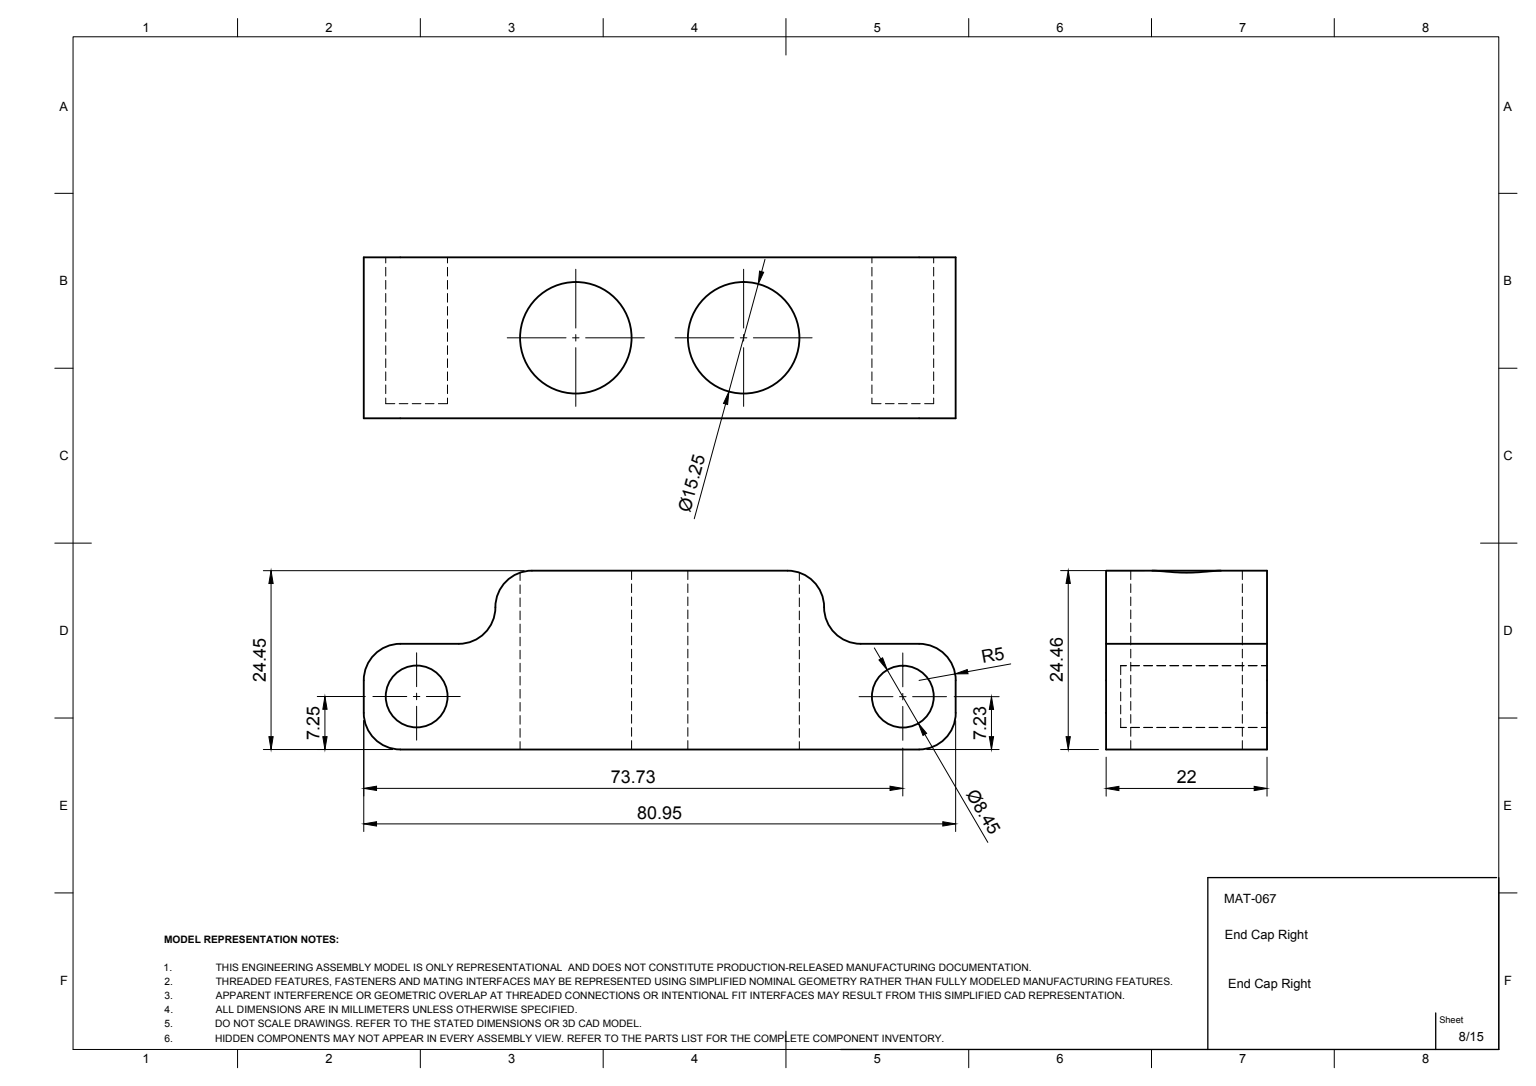
ISO-10303-21;
HEADER;
/* Generated by software containing ST-Developer
 * from STEP Tools, Inc. (www.steptools.com) 
 */

FILE_DESCRIPTION(
/* description */ ('CAx-IF Rec.Pracs.---Representation and Presentation of Product Manufa
cturing Information (PMI)---4.0---2014-10-13'),
/* implementation_level */ '2;1');

FILE_NAME(
/* name */ 'End Cap Right.step',
/* time_stamp */ '2026-10-24T16:02:03-07:00',
/* author */ (''),
/* organization */ (''),
/* preprocessor_version */ 'ST-DEVELOPER v20.2',
/* originating_system */ 'Autodesk Translation Framework v15.17.0.0',
/* authorisation */ '');

FILE_SCHEMA (('AP242_MANAGED_MODEL_BASED_3D_ENGINEERING_MIM_LF { 1 0 10303 442 2 1 4 }'));
ENDSEC;

DATA;
#10=MECHANICAL_DESIGN_GEOMETRIC_PRESENTATION_REPRESENTATION('',(#353),#6348);
#331=SHAPE_REPRESENTATION_RELATIONSHIP('SRR','None',#6482,#342);
#342=ADVANCED_BREP_SHAPE_REPRESENTATION('',(#364),#6330);
#353=STYLED_ITEM('',(#6603),#364);
#364=MANIFOLD_SOLID_BREP('Body1',#3392);
#379=B_SPLINE_CURVE_WITH_KNOTS('',3,(#5841,#5842,#5843,#5844,#5845,#5846),
 .UNSPECIFIED.,.F.,.F.,(4,2,4),(3.46797062946804,3.66737221611079,3.95578831781598),
 .UNSPECIFIED.);
#380=B_SPLINE_CURVE_WITH_KNOTS('',3,(#5847,#5848,#5849,#5850,#5851,#5852),
 .UNSPECIFIED.,.F.,.F.,(4,2,4),(3.95578831781598,4.24420441952117,4.44360600616391),
 .UNSPECIFIED.);
#381=B_SPLINE_CURVE_WITH_KNOTS('',3,(#5855,#5856,#5857,#5858,#5859,#5860,
#5861,#5862,#5863,#5864),.UNSPECIFIED.,.F.,.F.,(4,2,2,2,4),(3.46797062946804,
3.66737221611078,3.95578831781597,4.24420441952117,4.44360600616391),
 .UNSPECIFIED.);
#421=CYLINDRICAL_SURFACE('',#3690,0.004225);
#422=CYLINDRICAL_SURFACE('',#3694,0.004225);
#423=CYLINDRICAL_SURFACE('',#3717,0.005);
#424=CYLINDRICAL_SURFACE('',#3718,0.005);
#425=CYLINDRICAL_SURFACE('',#3719,0.005);
#426=CYLINDRICAL_SURFACE('',#3720,0.005);
#427=CYLINDRICAL_SURFACE('',#3725,0.007625);
#428=CYLINDRICAL_SURFACE('',#3726,0.007625);
#429=CYLINDRICAL_SURFACE('',#3727,0.005);
#430=CYLINDRICAL_SURFACE('',#3728,0.005);
#431=CYLINDRICAL_SURFACE('',#3729,0.005);
#432=CYLINDRICAL_SURFACE('',#3730,0.005);
#480=FACE_BOUND('',#960,.T.);
#481=FACE_BOUND('',#961,.T.);
#482=FACE_BOUND('',#967,.T.);
#483=FACE_BOUND('',#968,.T.);
#586=CIRCLE('',#3687,0.007625);
#587=CIRCLE('',#3688,0.007625);
#588=CIRCLE('',#3691,0.004225);
#589=CIRCLE('',#3692,0.004225);
#590=CIRCLE('',#3695,0.004225);
#591=CIRCLE('',#3696,0.004225);
#592=CIRCLE('',#3698,0.005);
#593=CIRCLE('',#3699,0.005);
#594=CIRCLE('',#3700,0.005);
#595=CIRCLE('',#3701,0.005);
#596=CIRCLE('',#3702,0.005);
#597=CIRCLE('',#3703,0.005);
#598=CIRCLE('',#3704,0.005);
#599=CIRCLE('',#3705,0.005);
#600=CIRCLE('',#3709,0.005);
#601=CIRCLE('',#3710,0.005);
#602=CIRCLE('',#3711,0.005);
#603=CIRCLE('',#3712,0.005);
#604=CIRCLE('',#3713,0.005);
#605=CIRCLE('',#3714,0.005);
#606=CIRCLE('',#3715,0.005);
#607=CIRCLE('',#3716,0.005);
#608=CIRCLE('',#3722,0.007625);
#609=CIRCLE('',#3723,0.007625);
#610=CIRCLE('',#3724,0.007625);
#770=FACE_OUTER_BOUND('',#957,.T.);
#771=FACE_OUTER_BOUND('',#958,.T.);
#772=FACE_OUTER_BOUND('',#959,.T.);
#773=FACE_OUTER_BOUND('',#962,.T.);
#774=FACE_OUTER_BOUND('',#963,.T.);
#775=FACE_OUTER_BOUND('',#964,.T.);
#776=FACE_OUTER_BOUND('',#965,.T.);
#777=FACE_OUTER_BOUND('',#966,.T.);
#778=FACE_OUTER_BOUND('',#969,.T.);
#779=FACE_OUTER_BOUND('',#970,.T.);
#780=FACE_OUTER_BOUND('',#971,.T.);
#781=FACE_OUTER_BOUND('',#972,.T.);
#782=FACE_OUTER_BOUND('',#973,.T.);
#783=FACE_OUTER_BOUND('',#974,.T.);
#784=FACE_OUTER_BOUND('',#975,.T.);
#785=FACE_OUTER_BOUND('',#976,.T.);
#786=FACE_OUTER_BOUND('',#977,.T.);
#787=FACE_OUTER_BOUND('',#978,.T.);
#788=FACE_OUTER_BOUND('',#979,.T.);
#789=FACE_OUTER_BOUND('',#980,.T.);
#790=FACE_OUTER_BOUND('',#981,.T.);
#791=FACE_OUTER_BOUND('',#982,.T.);
#957=EDGE_LOOP('',(#2723,#2724,#2725,#2726));
#958=EDGE_LOOP('',(#2727,#2728,#2729,#2730));
#959=EDGE_LOOP('',(#2731,#2732,#2733,#2734));
#960=EDGE_LOOP('',(#2735));
#961=EDGE_LOOP('',(#2736));
#962=EDGE_LOOP('',(#2737,#2738,#2739,#2740));
#963=EDGE_LOOP('',(#2741,#2742,#2743,#2744));
#964=EDGE_LOOP('',(#2745,#2746,#2747,#2748));
#965=EDGE_LOOP('',(#2749,#2750,#2751,#2752));
#966=EDGE_LOOP('',(#2753,#2754,#2755,#2756,#2757,#2758,#2759,#2760,#2761,
#2762,#2763,#2764,#2765,#2766));
#967=EDGE_LOOP('',(#2767));
#968=EDGE_LOOP('',(#2768));
#969=EDGE_LOOP('',(#2769));
#970=EDGE_LOOP('',(#2770));
#971=EDGE_LOOP('',(#2771,#2772,#2773,#2774,#2775,#2776,#2777,#2778,#2779,
#2780,#2781,#2782,#2783,#2784));
#972=EDGE_LOOP('',(#2785,#2786,#2787,#2788));
#973=EDGE_LOOP('',(#2789,#2790,#2791,#2792));
#974=EDGE_LOOP('',(#2793,#2794,#2795,#2796));
#975=EDGE_LOOP('',(#2797,#2798,#2799,#2800));
#976=EDGE_LOOP('',(#2801,#2802,#2803,#2804,#2805,#2806,#2807,#2808,#2809));
#977=EDGE_LOOP('',(#2810,#2811,#2812,#2813,#2814,#2815));
#978=EDGE_LOOP('',(#2816,#2817,#2818,#2819,#2820,#2821));
#979=EDGE_LOOP('',(#2822,#2823,#2824,#2825,#2826,#2827));
#980=EDGE_LOOP('',(#2828,#2829,#2830,#2831));
#981=EDGE_LOOP('',(#2832,#2833,#2834,#2835,#2836,#2837,#2838));
#982=EDGE_LOOP('',(#2839,#2840,#2841,#2842));
#1218=LINE('',#5733,#1451);
#1219=LINE('',#5735,#1452);
#1220=LINE('',#5737,#1453);
#1221=LINE('',#5738,#1454);
#1222=LINE('',#5742,#1455);
#1223=LINE('',#5744,#1456);
#1224=LINE('',#5746,#1457);
#1225=LINE('',#5747,#1458);
#1226=LINE('',#5751,#1459);
#1227=LINE('',#5753,#1460);
#1228=LINE('',#5755,#1461);
#1229=LINE('',#5756,#1462);
#1230=LINE('',#5764,#1463);
#1231=LINE('',#5766,#1464);
#1232=LINE('',#5768,#1465);
#1233=LINE('',#5769,#1466);
#1234=LINE('',#5774,#1467);
#1235=LINE('',#5779,#1468);
#1236=LINE('',#5781,#1469);
#1237=LINE('',#5783,#1470);
#1238=LINE('',#5784,#1471);
#1239=LINE('',#5789,#1472);
#1240=LINE('',#5794,#1473);
#1241=LINE('',#5817,#1474);
#1242=LINE('',#5827,#1475);
#1243=LINE('',#5830,#1476);
#1244=LINE('',#5832,#1477);
#1245=LINE('',#5837,#1478);
#1246=LINE('',#5840,#1479);
#1247=LINE('',#5854,#1480);
#1248=LINE('',#5866,#1481);
#1249=LINE('',#5869,#1482);
#1451=VECTOR('',#4448,1.);
#1452=VECTOR('',#4449,1.);
#1453=VECTOR('',#4450,1.);
#1454=VECTOR('',#4451,1.);
#1455=VECTOR('',#4454,1.);
#1456=VECTOR('',#4455,1.);
#1457=VECTOR('',#4456,1.);
#1458=VECTOR('',#4457,1.);
#1459=VECTOR('',#4460,1.);
#1460=VECTOR('',#4461,1.);
#1461=VECTOR('',#4462,1.);
#1462=VECTOR('',#4463,1.);
#1463=VECTOR('',#4470,1.);
#1464=VECTOR('',#4471,1.);
#1465=VECTOR('',#4472,1.);
#1466=VECTOR('',#4473,1.);
#1467=VECTOR('',#4478,0.004225);
#1468=VECTOR('',#4483,1.);
#1469=VECTOR('',#4484,1.);
#1470=VECTOR('',#4485,1.);
#1471=VECTOR('',#4486,1.);
#1472=VECTOR('',#4491,0.004225);
#1473=VECTOR('',#4496,1.);
#1474=VECTOR('',#4531,1.);
#1475=VECTOR('',#4546,1.);
#1476=VECTOR('',#4549,1.);
#1477=VECTOR('',#4550,1.);
#1478=VECTOR('',#4555,1.);
#1479=VECTOR('',#4558,0.007625);
#1480=VECTOR('',#4561,0.007625);
#1481=VECTOR('',#4564,1.);
#1482=VECTOR('',#4569,1.);
#1696=VERTEX_POINT('',#5731);
#1697=VERTEX_POINT('',#5732);
#1698=VERTEX_POINT('',#5734);
#1699=VERTEX_POINT('',#5736);
#1700=VERTEX_POINT('',#5740);
#1701=VERTEX_POINT('',#5741);
#1702=VERTEX_POINT('',#5743);
#1703=VERTEX_POINT('',#5745);
#1704=VERTEX_POINT('',#5749);
#1705=VERTEX_POINT('',#5750);
#1706=VERTEX_POINT('',#5752);
#1707=VERTEX_POINT('',#5754);
#1708=VERTEX_POINT('',#5757);
#1709=VERTEX_POINT('',#5759);
#1710=VERTEX_POINT('',#5762);
#1711=VERTEX_POINT('',#5763);
#1712=VERTEX_POINT('',#5765);
#1713=VERTEX_POINT('',#5767);
#1714=VERTEX_POINT('',#5771);
#1715=VERTEX_POINT('',#5773);
#1716=VERTEX_POINT('',#5777);
#1717=VERTEX_POINT('',#5778);
#1718=VERTEX_POINT('',#5780);
#1719=VERTEX_POINT('',#5782);
#1720=VERTEX_POINT('',#5786);
#1721=VERTEX_POINT('',#5788);
#1722=VERTEX_POINT('',#5792);
#1723=VERTEX_POINT('',#5793);
#1724=VERTEX_POINT('',#5795);
#1725=VERTEX_POINT('',#5802);
#1726=VERTEX_POINT('',#5812);
#1727=VERTEX_POINT('',#5814);
#1728=VERTEX_POINT('',#5816);
#1729=VERTEX_POINT('',#5818);
#1730=VERTEX_POINT('',#5826);
#1731=VERTEX_POINT('',#5828);
#1732=VERTEX_POINT('',#5831);
#1733=VERTEX_POINT('',#5833);
#1734=VERTEX_POINT('',#5835);
#1735=VERTEX_POINT('',#5839);
#2060=EDGE_CURVE('',#1696,#1697,#1218,.T.);
#2061=EDGE_CURVE('',#1698,#1697,#1219,.T.);
#2062=EDGE_CURVE('',#1699,#1698,#1220,.T.);
#2063=EDGE_CURVE('',#1696,#1699,#1221,.F.);
#2064=EDGE_CURVE('',#1700,#1701,#1222,.T.);
#2065=EDGE_CURVE('',#1702,#1700,#1223,.F.);
#2066=EDGE_CURVE('',#1702,#1703,#1224,.T.);
#2067=EDGE_CURVE('',#1701,#1703,#1225,.T.);
#2068=EDGE_CURVE('',#1704,#1705,#1226,.T.);
#2069=EDGE_CURVE('',#1706,#1705,#1227,.F.);
#2070=EDGE_CURVE('',#1707,#1706,#1228,.T.);
#2071=EDGE_CURVE('',#1704,#1707,#1229,.T.);
#2072=EDGE_CURVE('',#1708,#1708,#586,.T.);
#2073=EDGE_CURVE('',#1709,#1709,#587,.T.);
#2074=EDGE_CURVE('',#1710,#1711,#1230,.T.);
#2075=EDGE_CURVE('',#1712,#1711,#1231,.F.);
#2076=EDGE_CURVE('',#1713,#1712,#1232,.T.);
#2077=EDGE_CURVE('',#1710,#1713,#1233,.T.);
#2078=EDGE_CURVE('',#1714,#1714,#588,.T.);
#2079=EDGE_CURVE('',#1714,#1715,#1234,.T.);
#2080=EDGE_CURVE('',#1715,#1715,#589,.T.);
#2081=EDGE_CURVE('',#1716,#1717,#1235,.T.);
#2082=EDGE_CURVE('',#1718,#1716,#1236,.F.);
#2083=EDGE_CURVE('',#1718,#1719,#1237,.T.);
#2084=EDGE_CURVE('',#1717,#1719,#1238,.T.);
#2085=EDGE_CURVE('',#1720,#1720,#590,.T.);
#2086=EDGE_CURVE('',#1720,#1721,#1239,.T.);
#2087=EDGE_CURVE('',#1721,#1721,#591,.T.);
#2088=EDGE_CURVE('',#1722,#1723,#1240,.T.);
#2089=EDGE_CURVE('',#1724,#1722,#592,.F.);
#2090=EDGE_CURVE('',#1719,#1724,#593,.T.);
#2091=EDGE_CURVE('',#1703,#1718,#594,.F.);
#2092=EDGE_CURVE('',#1707,#1702,#595,.F.);
#2093=EDGE_CURVE('',#1713,#1706,#596,.F.);
#2094=EDGE_CURVE('',#1697,#1712,#597,.F.);
#2095=EDGE_CURVE('',#1725,#1696,#598,.T.);
#2096=EDGE_CURVE('',#1723,#1725,#599,.F.);
#2097=EDGE_CURVE('',#1711,#1698,#600,.T.);
#2098=EDGE_CURVE('',#1705,#1710,#601,.T.);
#2099=EDGE_CURVE('',#1700,#1704,#602,.T.);
#2100=EDGE_CURVE('',#1716,#1701,#603,.T.);
#2101=EDGE_CURVE('',#1726,#1717,#604,.F.);
#2102=EDGE_CURVE('',#1727,#1726,#605,.T.);
#2103=EDGE_CURVE('',#1727,#1728,#1241,.T.);
#2104=EDGE_CURVE('',#1729,#1728,#606,.T.);
#2105=EDGE_CURVE('',#1699,#1729,#607,.F.);
#2106=EDGE_CURVE('',#1730,#1727,#1242,.F.);
#2107=EDGE_CURVE('',#1730,#1731,#608,.T.);
#2108=EDGE_CURVE('',#1722,#1731,#1243,.F.);
#2109=EDGE_CURVE('',#1732,#1723,#1244,.T.);
#2110=EDGE_CURVE('',#1732,#1733,#609,.T.);
#2111=EDGE_CURVE('',#1733,#1734,#610,.T.);
#2112=EDGE_CURVE('',#1728,#1734,#1245,.T.);
#2113=EDGE_CURVE('',#1709,#1735,#1246,.T.);
#2114=EDGE_CURVE('',#1731,#1735,#379,.T.);
#2115=EDGE_CURVE('',#1735,#1730,#380,.T.);
#2116=EDGE_CURVE('',#1708,#1733,#1247,.T.);
#2117=EDGE_CURVE('',#1734,#1732,#381,.T.);
#2118=EDGE_CURVE('',#1725,#1729,#1248,.F.);
#2119=EDGE_CURVE('',#1726,#1724,#1249,.T.);
#2723=ORIENTED_EDGE('',*,*,#2060,.T.);
#2724=ORIENTED_EDGE('',*,*,#2061,.F.);
#2725=ORIENTED_EDGE('',*,*,#2062,.F.);
#2726=ORIENTED_EDGE('',*,*,#2063,.F.);
#2727=ORIENTED_EDGE('',*,*,#2064,.F.);
#2728=ORIENTED_EDGE('',*,*,#2065,.F.);
#2729=ORIENTED_EDGE('',*,*,#2066,.T.);
#2730=ORIENTED_EDGE('',*,*,#2067,.F.);
#2731=ORIENTED_EDGE('',*,*,#2068,.T.);
#2732=ORIENTED_EDGE('',*,*,#2069,.F.);
#2733=ORIENTED_EDGE('',*,*,#2070,.F.);
#2734=ORIENTED_EDGE('',*,*,#2071,.F.);
#2735=ORIENTED_EDGE('',*,*,#2072,.F.);
#2736=ORIENTED_EDGE('',*,*,#2073,.F.);
#2737=ORIENTED_EDGE('',*,*,#2074,.T.);
#2738=ORIENTED_EDGE('',*,*,#2075,.F.);
#2739=ORIENTED_EDGE('',*,*,#2076,.F.);
#2740=ORIENTED_EDGE('',*,*,#2077,.F.);
#2741=ORIENTED_EDGE('',*,*,#2078,.F.);
#2742=ORIENTED_EDGE('',*,*,#2079,.T.);
#2743=ORIENTED_EDGE('',*,*,#2080,.T.);
#2744=ORIENTED_EDGE('',*,*,#2079,.F.);
#2745=ORIENTED_EDGE('',*,*,#2081,.F.);
#2746=ORIENTED_EDGE('',*,*,#2082,.F.);
#2747=ORIENTED_EDGE('',*,*,#2083,.T.);
#2748=ORIENTED_EDGE('',*,*,#2084,.F.);
#2749=ORIENTED_EDGE('',*,*,#2085,.F.);
#2750=ORIENTED_EDGE('',*,*,#2086,.T.);
#2751=ORIENTED_EDGE('',*,*,#2087,.T.);
#2752=ORIENTED_EDGE('',*,*,#2086,.F.);
#2753=ORIENTED_EDGE('',*,*,#2088,.F.);
#2754=ORIENTED_EDGE('',*,*,#2089,.F.);
#2755=ORIENTED_EDGE('',*,*,#2090,.F.);
#2756=ORIENTED_EDGE('',*,*,#2083,.F.);
#2757=ORIENTED_EDGE('',*,*,#2091,.F.);
#2758=ORIENTED_EDGE('',*,*,#2066,.F.);
#2759=ORIENTED_EDGE('',*,*,#2092,.F.);
#2760=ORIENTED_EDGE('',*,*,#2070,.T.);
#2761=ORIENTED_EDGE('',*,*,#2093,.F.);
#2762=ORIENTED_EDGE('',*,*,#2076,.T.);
#2763=ORIENTED_EDGE('',*,*,#2094,.F.);
#2764=ORIENTED_EDGE('',*,*,#2060,.F.);
#2765=ORIENTED_EDGE('',*,*,#2095,.F.);
#2766=ORIENTED_EDGE('',*,*,#2096,.F.);
#2767=ORIENTED_EDGE('',*,*,#2080,.F.);
#2768=ORIENTED_EDGE('',*,*,#2087,.F.);
#2769=ORIENTED_EDGE('',*,*,#2085,.T.);
#2770=ORIENTED_EDGE('',*,*,#2078,.T.);
#2771=ORIENTED_EDGE('',*,*,#2062,.T.);
#2772=ORIENTED_EDGE('',*,*,#2097,.F.);
#2773=ORIENTED_EDGE('',*,*,#2074,.F.);
#2774=ORIENTED_EDGE('',*,*,#2098,.F.);
#2775=ORIENTED_EDGE('',*,*,#2068,.F.);
#2776=ORIENTED_EDGE('',*,*,#2099,.F.);
#2777=ORIENTED_EDGE('',*,*,#2064,.T.);
#2778=ORIENTED_EDGE('',*,*,#2100,.F.);
#2779=ORIENTED_EDGE('',*,*,#2081,.T.);
#2780=ORIENTED_EDGE('',*,*,#2101,.F.);
#2781=ORIENTED_EDGE('',*,*,#2102,.F.);
#2782=ORIENTED_EDGE('',*,*,#2103,.T.);
#2783=ORIENTED_EDGE('',*,*,#2104,.F.);
#2784=ORIENTED_EDGE('',*,*,#2105,.F.);
#2785=ORIENTED_EDGE('',*,*,#2100,.T.);
#2786=ORIENTED_EDGE('',*,*,#2067,.T.);
#2787=ORIENTED_EDGE('',*,*,#2091,.T.);
#2788=ORIENTED_EDGE('',*,*,#2082,.T.);
#2789=ORIENTED_EDGE('',*,*,#2099,.T.);
#2790=ORIENTED_EDGE('',*,*,#2071,.T.);
#2791=ORIENTED_EDGE('',*,*,#2092,.T.);
#2792=ORIENTED_EDGE('',*,*,#2065,.T.);
#2793=ORIENTED_EDGE('',*,*,#2098,.T.);
#2794=ORIENTED_EDGE('',*,*,#2077,.T.);
#2795=ORIENTED_EDGE('',*,*,#2093,.T.);
#2796=ORIENTED_EDGE('',*,*,#2069,.T.);
#2797=ORIENTED_EDGE('',*,*,#2097,.T.);
#2798=ORIENTED_EDGE('',*,*,#2061,.T.);
#2799=ORIENTED_EDGE('',*,*,#2094,.T.);
#2800=ORIENTED_EDGE('',*,*,#2075,.T.);
#2801=ORIENTED_EDGE('',*,*,#2103,.F.);
#2802=ORIENTED_EDGE('',*,*,#2106,.F.);
#2803=ORIENTED_EDGE('',*,*,#2107,.T.);
#2804=ORIENTED_EDGE('',*,*,#2108,.F.);
#2805=ORIENTED_EDGE('',*,*,#2088,.T.);
#2806=ORIENTED_EDGE('',*,*,#2109,.F.);
#2807=ORIENTED_EDGE('',*,*,#2110,.T.);
#2808=ORIENTED_EDGE('',*,*,#2111,.T.);
#2809=ORIENTED_EDGE('',*,*,#2112,.F.);
#2810=ORIENTED_EDGE('',*,*,#2073,.T.);
#2811=ORIENTED_EDGE('',*,*,#2113,.T.);
#2812=ORIENTED_EDGE('',*,*,#2114,.F.);
#2813=ORIENTED_EDGE('',*,*,#2107,.F.);
#2814=ORIENTED_EDGE('',*,*,#2115,.F.);
#2815=ORIENTED_EDGE('',*,*,#2113,.F.);
#2816=ORIENTED_EDGE('',*,*,#2072,.T.);
#2817=ORIENTED_EDGE('',*,*,#2116,.T.);
#2818=ORIENTED_EDGE('',*,*,#2110,.F.);
#2819=ORIENTED_EDGE('',*,*,#2117,.F.);
#2820=ORIENTED_EDGE('',*,*,#2111,.F.);
#2821=ORIENTED_EDGE('',*,*,#2116,.F.);
#2822=ORIENTED_EDGE('',*,*,#2112,.T.);
#2823=ORIENTED_EDGE('',*,*,#2117,.T.);
#2824=ORIENTED_EDGE('',*,*,#2109,.T.);
#2825=ORIENTED_EDGE('',*,*,#2096,.T.);
#2826=ORIENTED_EDGE('',*,*,#2118,.T.);
#2827=ORIENTED_EDGE('',*,*,#2104,.T.);
#2828=ORIENTED_EDGE('',*,*,#2105,.T.);
#2829=ORIENTED_EDGE('',*,*,#2118,.F.);
#2830=ORIENTED_EDGE('',*,*,#2095,.T.);
#2831=ORIENTED_EDGE('',*,*,#2063,.T.);
#2832=ORIENTED_EDGE('',*,*,#2119,.T.);
#2833=ORIENTED_EDGE('',*,*,#2089,.T.);
#2834=ORIENTED_EDGE('',*,*,#2108,.T.);
#2835=ORIENTED_EDGE('',*,*,#2114,.T.);
#2836=ORIENTED_EDGE('',*,*,#2115,.T.);
#2837=ORIENTED_EDGE('',*,*,#2106,.T.);
#2838=ORIENTED_EDGE('',*,*,#2102,.T.);
#2839=ORIENTED_EDGE('',*,*,#2101,.T.);
#2840=ORIENTED_EDGE('',*,*,#2084,.T.);
#2841=ORIENTED_EDGE('',*,*,#2090,.T.);
#2842=ORIENTED_EDGE('',*,*,#2119,.F.);
#3177=PLANE('',#3684);
#3178=PLANE('',#3685);
#3179=PLANE('',#3686);
#3180=PLANE('',#3689);
#3181=PLANE('',#3693);
#3182=PLANE('',#3697);
#3183=PLANE('',#3706);
#3184=PLANE('',#3707);
#3185=PLANE('',#3708);
#3186=PLANE('',#3721);
#3293=ADVANCED_FACE('',(#770),#3177,.T.);
#3294=ADVANCED_FACE('',(#771),#3178,.T.);
#3295=ADVANCED_FACE('',(#772,#480,#481),#3179,.F.);
#3296=ADVANCED_FACE('',(#773),#3180,.F.);
#3297=ADVANCED_FACE('',(#774),#421,.F.);
#3298=ADVANCED_FACE('',(#775),#3181,.T.);
#3299=ADVANCED_FACE('',(#776),#422,.F.);
#3300=ADVANCED_FACE('',(#777,#482,#483),#3182,.F.);
#3301=ADVANCED_FACE('',(#778),#3183,.F.);
#3302=ADVANCED_FACE('',(#779),#3184,.F.);
#3303=ADVANCED_FACE('',(#780),#3185,.T.);
#3304=ADVANCED_FACE('',(#781),#423,.T.);
#3305=ADVANCED_FACE('',(#782),#424,.T.);
#3306=ADVANCED_FACE('',(#783),#425,.T.);
#3307=ADVANCED_FACE('',(#784),#426,.T.);
#3308=ADVANCED_FACE('',(#785),#3186,.T.);
#3309=ADVANCED_FACE('',(#786),#427,.F.);
#3310=ADVANCED_FACE('',(#787),#428,.F.);
#3311=ADVANCED_FACE('',(#788),#429,.T.);
#3312=ADVANCED_FACE('',(#789),#430,.F.);
#3313=ADVANCED_FACE('',(#790),#431,.T.);
#3314=ADVANCED_FACE('',(#791),#432,.F.);
#3392=CLOSED_SHELL('',(#3293,#3294,#3295,#3296,#3297,#3298,#3299,#3300,
#3301,#3302,#3303,#3304,#3305,#3306,#3307,#3308,#3309,#3310,#3311,#3312,
#3313,#3314));
#3683=AXIS2_PLACEMENT_3D('',#5729,#4444,#4445);
#3684=AXIS2_PLACEMENT_3D('',#5730,#4446,#4447);
#3685=AXIS2_PLACEMENT_3D('',#5739,#4452,#4453);
#3686=AXIS2_PLACEMENT_3D('',#5748,#4458,#4459);
#3687=AXIS2_PLACEMENT_3D('',#5758,#4464,#4465);
#3688=AXIS2_PLACEMENT_3D('',#5760,#4466,#4467);
#3689=AXIS2_PLACEMENT_3D('',#5761,#4468,#4469);
#3690=AXIS2_PLACEMENT_3D('',#5770,#4474,#4475);
#3691=AXIS2_PLACEMENT_3D('',#5772,#4476,#4477);
#3692=AXIS2_PLACEMENT_3D('',#5775,#4479,#4480);
#3693=AXIS2_PLACEMENT_3D('',#5776,#4481,#4482);
#3694=AXIS2_PLACEMENT_3D('',#5785,#4487,#4488);
#3695=AXIS2_PLACEMENT_3D('',#5787,#4489,#4490);
#3696=AXIS2_PLACEMENT_3D('',#5790,#4492,#4493);
#3697=AXIS2_PLACEMENT_3D('',#5791,#4494,#4495);
#3698=AXIS2_PLACEMENT_3D('',#5796,#4497,#4498);
#3699=AXIS2_PLACEMENT_3D('',#5797,#4499,#4500);
#3700=AXIS2_PLACEMENT_3D('',#5798,#4501,#4502);
#3701=AXIS2_PLACEMENT_3D('',#5799,#4503,#4504);
#3702=AXIS2_PLACEMENT_3D('',#5800,#4505,#4506);
#3703=AXIS2_PLACEMENT_3D('',#5801,#4507,#4508);
#3704=AXIS2_PLACEMENT_3D('',#5803,#4509,#4510);
#3705=AXIS2_PLACEMENT_3D('',#5804,#4511,#4512);
#3706=AXIS2_PLACEMENT_3D('',#5805,#4513,#4514);
#3707=AXIS2_PLACEMENT_3D('',#5806,#4515,#4516);
#3708=AXIS2_PLACEMENT_3D('',#5807,#4517,#4518);
#3709=AXIS2_PLACEMENT_3D('',#5808,#4519,#4520);
#3710=AXIS2_PLACEMENT_3D('',#5809,#4521,#4522);
#3711=AXIS2_PLACEMENT_3D('',#5810,#4523,#4524);
#3712=AXIS2_PLACEMENT_3D('',#5811,#4525,#4526);
#3713=AXIS2_PLACEMENT_3D('',#5813,#4527,#4528);
#3714=AXIS2_PLACEMENT_3D('',#5815,#4529,#4530);
#3715=AXIS2_PLACEMENT_3D('',#5819,#4532,#4533);
#3716=AXIS2_PLACEMENT_3D('',#5820,#4534,#4535);
#3717=AXIS2_PLACEMENT_3D('',#5821,#4536,#4537);
#3718=AXIS2_PLACEMENT_3D('',#5822,#4538,#4539);
#3719=AXIS2_PLACEMENT_3D('',#5823,#4540,#4541);
#3720=AXIS2_PLACEMENT_3D('',#5824,#4542,#4543);
#3721=AXIS2_PLACEMENT_3D('',#5825,#4544,#4545);
#3722=AXIS2_PLACEMENT_3D('',#5829,#4547,#4548);
#3723=AXIS2_PLACEMENT_3D('',#5834,#4551,#4552);
#3724=AXIS2_PLACEMENT_3D('',#5836,#4553,#4554);
#3725=AXIS2_PLACEMENT_3D('',#5838,#4556,#4557);
#3726=AXIS2_PLACEMENT_3D('',#5853,#4559,#4560);
#3727=AXIS2_PLACEMENT_3D('',#5865,#4562,#4563);
#3728=AXIS2_PLACEMENT_3D('',#5867,#4565,#4566);
#3729=AXIS2_PLACEMENT_3D('',#5868,#4567,#4568);
#3730=AXIS2_PLACEMENT_3D('',#5870,#4570,#4571);
#4444=DIRECTION('axis',(0.,0.,1.));
#4445=DIRECTION('refdir',(1.,0.,0.));
#4446=DIRECTION('center_axis',(0.,-1.,8.57182693503055E-17));
#4447=DIRECTION('ref_axis',(0.,-8.57182693503055E-17,-1.));
#4448=DIRECTION('',(0.,-8.57182693503055E-17,-1.));
#4449=DIRECTION('',(-1.,0.,0.));
#4450=DIRECTION('',(0.,-8.57182693503055E-17,-1.));
#4451=DIRECTION('',(-1.,0.,0.));
#4452=DIRECTION('center_axis',(0.,0.,1.));
#4453=DIRECTION('ref_axis',(-1.,0.,0.));
#4454=DIRECTION('',(0.,-1.,0.));
#4455=DIRECTION('',(-1.,0.,0.));
#4456=DIRECTION('',(0.,-1.,0.));
#4457=DIRECTION('',(-1.,0.,0.));
#4458=DIRECTION('center_axis',(0.,-1.,6.42887020127291E-17));
#4459=DIRECTION('ref_axis',(0.,-6.42887020127291E-17,-1.));
#4460=DIRECTION('',(0.,-6.42887020127291E-17,-1.));
#4461=DIRECTION('',(-1.,0.,0.));
#4462=DIRECTION('',(0.,-6.42887020127291E-17,-1.));
#4463=DIRECTION('',(-1.,0.,0.));
#4464=DIRECTION('center_axis',(0.,1.,-6.42887020127291E-17));
#4465=DIRECTION('ref_axis',(0.,-6.42887020127291E-17,-1.));
#4466=DIRECTION('center_axis',(0.,1.,-6.42887020127291E-17));
#4467=DIRECTION('ref_axis',(0.,-6.42887020127291E-17,-1.));
#4468=DIRECTION('center_axis',(0.,0.,1.));
#4469=DIRECTION('ref_axis',(-1.,0.,0.));
#4470=DIRECTION('',(0.,-1.,0.));
#4471=DIRECTION('',(-1.,0.,0.));
#4472=DIRECTION('',(0.,-1.,0.));
#4473=DIRECTION('',(-1.,0.,0.));
#4474=DIRECTION('center_axis',(-1.,0.,0.));
#4475=DIRECTION('ref_axis',(0.,0.,-1.));
#4476=DIRECTION('center_axis',(-1.,0.,0.));
#4477=DIRECTION('ref_axis',(0.,0.,1.));
#4478=DIRECTION('',(-1.,0.,0.));
#4479=DIRECTION('center_axis',(-1.,0.,0.));
#4480=DIRECTION('ref_axis',(0.,0.,1.));
#4481=DIRECTION('center_axis',(0.,-1.,8.57182693503055E-17));
#4482=DIRECTION('ref_axis',(0.,-8.57182693503055E-17,-1.));
#4483=DIRECTION('',(0.,-8.57182693503055E-17,-1.));
#4484=DIRECTION('',(-1.,0.,0.));
#4485=DIRECTION('',(0.,-8.57182693503055E-17,-1.));
#4486=DIRECTION('',(-1.,0.,0.));
#4487=DIRECTION('center_axis',(-1.,0.,0.));
#4488=DIRECTION('ref_axis',(0.,0.,-1.));
#4489=DIRECTION('center_axis',(-1.,0.,0.));
#4490=DIRECTION('ref_axis',(0.,0.,1.));
#4491=DIRECTION('',(-1.,0.,0.));
#4492=DIRECTION('center_axis',(-1.,0.,0.));
#4493=DIRECTION('ref_axis',(0.,0.,1.));
#4494=DIRECTION('center_axis',(1.,0.,0.));
#4495=DIRECTION('ref_axis',(0.,-1.,0.));
#4496=DIRECTION('',(0.,-8.57182693503055E-17,-1.));
#4497=DIRECTION('center_axis',(-1.,0.,0.));
#4498=DIRECTION('ref_axis',(0.,0.,1.));
#4499=DIRECTION('center_axis',(-1.,0.,0.));
#4500=DIRECTION('ref_axis',(0.,0.,1.));
#4501=DIRECTION('center_axis',(-1.,0.,0.));
#4502=DIRECTION('ref_axis',(0.,0.,1.));
#4503=DIRECTION('center_axis',(-1.,0.,0.));
#4504=DIRECTION('ref_axis',(0.,0.,1.));
#4505=DIRECTION('center_axis',(-1.,0.,0.));
#4506=DIRECTION('ref_axis',(0.,0.,1.));
#4507=DIRECTION('center_axis',(-1.,0.,0.));
#4508=DIRECTION('ref_axis',(0.,0.,1.));
#4509=DIRECTION('center_axis',(-1.,0.,0.));
#4510=DIRECTION('ref_axis',(0.,0.,1.));
#4511=DIRECTION('center_axis',(-1.,0.,0.));
#4512=DIRECTION('ref_axis',(0.,0.,1.));
#4513=DIRECTION('center_axis',(1.,0.,0.));
#4514=DIRECTION('ref_axis',(0.,-1.,0.));
#4515=DIRECTION('center_axis',(1.,0.,0.));
#4516=DIRECTION('ref_axis',(0.,-1.,0.));
#4517=DIRECTION('center_axis',(1.,0.,0.));
#4518=DIRECTION('ref_axis',(0.,-1.,0.));
#4519=DIRECTION('center_axis',(-1.,0.,0.));
#4520=DIRECTION('ref_axis',(0.,0.,1.));
#4521=DIRECTION('center_axis',(-1.,0.,0.));
#4522=DIRECTION('ref_axis',(0.,0.,1.));
#4523=DIRECTION('center_axis',(-1.,0.,0.));
#4524=DIRECTION('ref_axis',(0.,0.,1.));
#4525=DIRECTION('center_axis',(-1.,0.,0.));
#4526=DIRECTION('ref_axis',(0.,0.,1.));
#4527=DIRECTION('center_axis',(-1.,0.,0.));
#4528=DIRECTION('ref_axis',(0.,0.,1.));
#4529=DIRECTION('center_axis',(-1.,0.,0.));
#4530=DIRECTION('ref_axis',(0.,0.,1.));
#4531=DIRECTION('',(0.,-8.57182693503055E-17,-1.));
#4532=DIRECTION('center_axis',(-1.,0.,0.));
#4533=DIRECTION('ref_axis',(0.,0.,1.));
#4534=DIRECTION('center_axis',(-1.,0.,0.));
#4535=DIRECTION('ref_axis',(0.,0.,1.));
#4536=DIRECTION('center_axis',(-1.,0.,0.));
#4537=DIRECTION('ref_axis',(0.,0.,-1.));
#4538=DIRECTION('center_axis',(1.,0.,0.));
#4539=DIRECTION('ref_axis',(0.,0.,1.));
#4540=DIRECTION('center_axis',(-1.,0.,0.));
#4541=DIRECTION('ref_axis',(0.,0.,-1.));
#4542=DIRECTION('center_axis',(1.,0.,0.));
#4543=DIRECTION('ref_axis',(0.,0.,1.));
#4544=DIRECTION('center_axis',(0.,-1.,8.57182693503055E-17));
#4545=DIRECTION('ref_axis',(-1.,0.,0.));
#4546=DIRECTION('',(-1.,0.,0.));
#4547=DIRECTION('center_axis',(0.,1.,-8.57182693503055E-17));
#4548=DIRECTION('ref_axis',(0.,-8.57182693503055E-17,-1.));
#4549=DIRECTION('',(-1.,0.,0.));
#4550=DIRECTION('',(-1.,0.,0.));
#4551=DIRECTION('center_axis',(0.,1.,-8.57182693503055E-17));
#4552=DIRECTION('ref_axis',(0.,-8.57182693503055E-17,-1.));
#4553=DIRECTION('center_axis',(0.,1.,-8.57182693503055E-17));
#4554=DIRECTION('ref_axis',(0.,-8.57182693503055E-17,-1.));
#4555=DIRECTION('',(-1.,0.,0.));
#4556=DIRECTION('center_axis',(0.,-1.,8.57182693503055E-17));
#4557=DIRECTION('ref_axis',(0.,-8.57182693503055E-17,-1.));
#4558=DIRECTION('',(0.,-1.,8.57182693503055E-17));
#4559=DIRECTION('center_axis',(0.,-1.,8.57182693503055E-17));
#4560=DIRECTION('ref_axis',(0.,-8.57182693503055E-17,-1.));
#4561=DIRECTION('',(0.,-1.,8.57182693503055E-17));
#4562=DIRECTION('center_axis',(1.,0.,0.));
#4563=DIRECTION('ref_axis',(0.,0.,1.));
#4564=DIRECTION('',(-1.,0.,0.));
#4565=DIRECTION('center_axis',(-1.,0.,0.));
#4566=DIRECTION('ref_axis',(0.,0.,-1.));
#4567=DIRECTION('center_axis',(-1.,0.,0.));
#4568=DIRECTION('ref_axis',(0.,0.,-1.));
#4569=DIRECTION('',(-1.,0.,0.));
#4570=DIRECTION('center_axis',(1.,0.,0.));
#4571=DIRECTION('ref_axis',(0.,0.,1.));
#5729=CARTESIAN_POINT('',(0.,0.,0.));
#5730=CARTESIAN_POINT('Origin',(0.06655,-0.0172,0.02565));
#5731=CARTESIAN_POINT('',(0.04655,-0.0172,-0.001825));
#5732=CARTESIAN_POINT('',(0.04655,-0.0172,-0.009825));
#5733=CARTESIAN_POINT('',(0.04655,-0.0172,0.02565));
#5734=CARTESIAN_POINT('',(0.06855,-0.0172,-0.009825));
#5735=CARTESIAN_POINT('',(0.04655,-0.0172,-0.009825));
#5736=CARTESIAN_POINT('',(0.06855,-0.0172,-0.001825));
#5737=CARTESIAN_POINT('',(0.06855,-0.0172,0.02565));
#5738=CARTESIAN_POINT('',(0.06655,-0.0172,-0.001825));
#5739=CARTESIAN_POINT('Origin',(0.06655,-0.009975,0.066125));
#5740=CARTESIAN_POINT('',(0.06855,-0.00775,0.066125));
#5741=CARTESIAN_POINT('',(0.06855,-0.0122,0.066125));
#5742=CARTESIAN_POINT('',(0.06855,-0.009975,0.066125));
#5743=CARTESIAN_POINT('',(0.04655,-0.00775,0.066125));
#5744=CARTESIAN_POINT('',(0.06855,-0.00775,0.066125));
#5745=CARTESIAN_POINT('',(0.04655,-0.0122,0.066125));
#5746=CARTESIAN_POINT('',(0.04655,-0.009975,0.066125));
#5747=CARTESIAN_POINT('',(0.06655,-0.0122,0.066125));
#5748=CARTESIAN_POINT('Origin',(0.06655,-0.00275,0.02565));
#5749=CARTESIAN_POINT('',(0.06855,-0.00275,0.061125));
#5750=CARTESIAN_POINT('',(0.06855,-0.00275,-0.009825));
#5751=CARTESIAN_POINT('',(0.06855,-0.00275,0.02565));
#5752=CARTESIAN_POINT('',(0.04655,-0.00275,-0.009825));
#5753=CARTESIAN_POINT('',(0.06655,-0.00275,-0.009825));
#5754=CARTESIAN_POINT('',(0.04655,-0.00275,0.061125));
#5755=CARTESIAN_POINT('',(0.04655,-0.00275,0.02565));
#5756=CARTESIAN_POINT('',(0.04655,-0.00275,0.061125));
#5757=CARTESIAN_POINT('',(0.05755,-0.00275,0.0218));
#5758=CARTESIAN_POINT('Origin',(0.05755,-0.00275,0.014175));
#5759=CARTESIAN_POINT('',(0.05755,-0.00275,0.04475));
#5760=CARTESIAN_POINT('Origin',(0.05755,-0.00275,0.037125));
#5761=CARTESIAN_POINT('Origin',(0.06655,-0.009975,-0.014825));
#5762=CARTESIAN_POINT('',(0.06855,-0.00775,-0.014825));
#5763=CARTESIAN_POINT('',(0.06855,-0.0122,-0.014825));
#5764=CARTESIAN_POINT('',(0.06855,-0.009975,-0.014825));
#5765=CARTESIAN_POINT('',(0.04655,-0.0122,-0.014825));
#5766=CARTESIAN_POINT('',(0.06855,-0.0122,-0.014825));
#5767=CARTESIAN_POINT('',(0.04655,-0.00775,-0.014825));
#5768=CARTESIAN_POINT('',(0.04655,-0.009975,-0.014825));
#5769=CARTESIAN_POINT('',(0.06655,-0.00775,-0.014825));
#5770=CARTESIAN_POINT('Origin',(0.06655,-0.009975,-0.0076));
#5771=CARTESIAN_POINT('',(0.06655,-0.009975,-0.003375));
#5772=CARTESIAN_POINT('Origin',(0.06655,-0.009975,-0.0076));
#5773=CARTESIAN_POINT('',(0.04655,-0.009975,-0.003375));
#5774=CARTESIAN_POINT('',(0.06655,-0.009975,-0.003375));
#5775=CARTESIAN_POINT('Origin',(0.04655,-0.009975,-0.0076));
#5776=CARTESIAN_POINT('Origin',(0.06655,-0.0172,0.02565));
#5777=CARTESIAN_POINT('',(0.06855,-0.0172,0.061125));
#5778=CARTESIAN_POINT('',(0.06855,-0.0172,0.053125));
#5779=CARTESIAN_POINT('',(0.06855,-0.0172,0.02565));
#5780=CARTESIAN_POINT('',(0.04655,-0.0172,0.061125));
#5781=CARTESIAN_POINT('',(0.06655,-0.0172,0.061125));
#5782=CARTESIAN_POINT('',(0.04655,-0.0172,0.053125));
#5783=CARTESIAN_POINT('',(0.04655,-0.0172,0.02565));
#5784=CARTESIAN_POINT('',(0.04655,-0.0172,0.053125));
#5785=CARTESIAN_POINT('Origin',(0.06655,-0.01,0.0589));
#5786=CARTESIAN_POINT('',(0.06655,-0.01,0.063125));
#5787=CARTESIAN_POINT('Origin',(0.06655,-0.01,0.0589));
#5788=CARTESIAN_POINT('',(0.04655,-0.01,0.063125));
#5789=CARTESIAN_POINT('',(0.06655,-0.01,0.063125));
#5790=CARTESIAN_POINT('Origin',(0.04655,-0.01,0.0589));
#5791=CARTESIAN_POINT('Origin',(0.04655,0.,0.02565));
#5792=CARTESIAN_POINT('',(0.04655,-0.0272,0.043125));
#5793=CARTESIAN_POINT('',(0.04655,-0.0272,0.008175));
#5794=CARTESIAN_POINT('',(0.04655,-0.0272,0.02565));
#5795=CARTESIAN_POINT('',(0.04655,-0.0222,0.048125));
#5796=CARTESIAN_POINT('Origin',(0.04655,-0.0222,0.043125));
#5797=CARTESIAN_POINT('Origin',(0.04655,-0.0222,0.053125));
#5798=CARTESIAN_POINT('Origin',(0.04655,-0.0122,0.061125));
#5799=CARTESIAN_POINT('Origin',(0.04655,-0.00775,0.061125));
#5800=CARTESIAN_POINT('Origin',(0.04655,-0.00775,-0.009825));
#5801=CARTESIAN_POINT('Origin',(0.04655,-0.0122,-0.009825));
#5802=CARTESIAN_POINT('',(0.04655,-0.0222,0.003175));
#5803=CARTESIAN_POINT('Origin',(0.04655,-0.0222,-0.001825));
#5804=CARTESIAN_POINT('Origin',(0.04655,-0.0222,0.008175));
#5805=CARTESIAN_POINT('Origin',(0.06655,-0.009975,0.02565));
#5806=CARTESIAN_POINT('Origin',(0.06655,-0.009975,0.02565));
#5807=CARTESIAN_POINT('Origin',(0.06855,-0.009975,0.02565));
#5808=CARTESIAN_POINT('Origin',(0.06855,-0.0122,-0.009825));
#5809=CARTESIAN_POINT('Origin',(0.06855,-0.00775,-0.009825));
#5810=CARTESIAN_POINT('Origin',(0.06855,-0.00775,0.061125));
#5811=CARTESIAN_POINT('Origin',(0.06855,-0.0122,0.061125));
#5812=CARTESIAN_POINT('',(0.06855,-0.0222,0.048125));
#5813=CARTESIAN_POINT('Origin',(0.06855,-0.0222,0.053125));
#5814=CARTESIAN_POINT('',(0.06855,-0.0272,0.043125));
#5815=CARTESIAN_POINT('Origin',(0.06855,-0.0222,0.043125));
#5816=CARTESIAN_POINT('',(0.06855,-0.0272,0.008175));
#5817=CARTESIAN_POINT('',(0.06855,-0.0272,0.02565));
#5818=CARTESIAN_POINT('',(0.06855,-0.0222,0.003175));
#5819=CARTESIAN_POINT('Origin',(0.06855,-0.0222,0.008175));
#5820=CARTESIAN_POINT('Origin',(0.06855,-0.0222,-0.001825));
#5821=CARTESIAN_POINT('Origin',(0.06655,-0.0122,0.061125));
#5822=CARTESIAN_POINT('Origin',(0.06655,-0.00775,0.061125));
#5823=CARTESIAN_POINT('Origin',(0.06655,-0.00775,-0.009825));
#5824=CARTESIAN_POINT('Origin',(0.06655,-0.0122,-0.009825));
#5825=CARTESIAN_POINT('Origin',(0.05755,-0.0272,0.02565));
#5826=CARTESIAN_POINT('',(0.0622553825561797,-0.0272,0.043125));
#5827=CARTESIAN_POINT('',(0.05755,-0.0272,0.043125));
#5828=CARTESIAN_POINT('',(0.0528446174438203,-0.0272,0.043125));
#5829=CARTESIAN_POINT('Origin',(0.05755,-0.0272,0.037125));
#5830=CARTESIAN_POINT('',(0.05755,-0.0272,0.043125));
#5831=CARTESIAN_POINT('',(0.0528446174438203,-0.0272,0.008175));
#5832=CARTESIAN_POINT('',(0.04655,-0.0272,0.008175));
#5833=CARTESIAN_POINT('',(0.05755,-0.0272,0.0218));
#5834=CARTESIAN_POINT('Origin',(0.05755,-0.0272,0.014175));
#5835=CARTESIAN_POINT('',(0.0622553825561797,-0.0272,0.008175));
#5836=CARTESIAN_POINT('Origin',(0.05755,-0.0272,0.014175));
#5837=CARTESIAN_POINT('',(0.04655,-0.0272,0.008175));
#5838=CARTESIAN_POINT('Origin',(0.05755,-0.0022,0.037125));
#5839=CARTESIAN_POINT('',(0.05755,-0.0269285700798444,0.04475));
#5840=CARTESIAN_POINT('',(0.05755,-0.0022,0.04475));
#5841=CARTESIAN_POINT('Ctrl Pts',(0.0528446174438203,-0.0272,0.043125));
#5842=CARTESIAN_POINT('Ctrl Pts',(0.0533814087034594,-0.0272,0.0435459680382359));
#5843=CARTESIAN_POINT('Ctrl Pts',(0.0539899057191737,-0.027146490983882,
0.0439040351600042));
#5844=CARTESIAN_POINT('Ctrl Pts',(0.0555707240629267,-0.0270066019492738,
0.0445577665669935));
#5845=CARTESIAN_POINT('Ctrl Pts',(0.056588612994316,-0.0269285700798444,
0.04475));
#5846=CARTESIAN_POINT('Ctrl Pts',(0.05755,-0.0269285700798444,0.04475));
#5847=CARTESIAN_POINT('Ctrl Pts',(0.05755,-0.0269285700798444,0.04475));
#5848=CARTESIAN_POINT('Ctrl Pts',(0.058511387005684,-0.0269285700798444,
0.04475));
#5849=CARTESIAN_POINT('Ctrl Pts',(0.0595292759370733,-0.0270066019492738,
0.0445577665669935));
#5850=CARTESIAN_POINT('Ctrl Pts',(0.0611100942808263,-0.027146490983882,
0.0439040351600042));
#5851=CARTESIAN_POINT('Ctrl Pts',(0.0617185912965407,-0.0272,0.0435459680382359));
#5852=CARTESIAN_POINT('Ctrl Pts',(0.0622553825561797,-0.0272,0.043125));
#5853=CARTESIAN_POINT('Origin',(0.05755,-0.0022,0.014175));
#5854=CARTESIAN_POINT('',(0.05755,-0.0022,0.0218));
#5855=CARTESIAN_POINT('Ctrl Pts',(0.0622553825561797,-0.0272,0.00817500000000001));
#5856=CARTESIAN_POINT('Ctrl Pts',(0.0617185912965407,-0.0272,0.00775403196176415));
#5857=CARTESIAN_POINT('Ctrl Pts',(0.0611100942808263,-0.027146490983882,
0.00739596483999584));
#5858=CARTESIAN_POINT('Ctrl Pts',(0.0595292759370733,-0.0270066019492738,
0.00674223343300649));
#5859=CARTESIAN_POINT('Ctrl Pts',(0.058511387005684,-0.0269285700798444,
0.00655));
#5860=CARTESIAN_POINT('Ctrl Pts',(0.056588612994316,-0.0269285700798444,
0.00655));
#5861=CARTESIAN_POINT('Ctrl Pts',(0.0555707240629267,-0.0270066019492738,
0.00674223343300649));
#5862=CARTESIAN_POINT('Ctrl Pts',(0.0539899057191737,-0.027146490983882,
0.00739596483999584));
#5863=CARTESIAN_POINT('Ctrl Pts',(0.0533814087034593,-0.0272,0.00775403196176414));
#5864=CARTESIAN_POINT('Ctrl Pts',(0.0528446174438203,-0.0272,0.00817500000000001));
#5865=CARTESIAN_POINT('Origin',(0.05755,-0.0222,0.008175));
#5866=CARTESIAN_POINT('',(0.06855,-0.0222,0.003175));
#5867=CARTESIAN_POINT('Origin',(0.05755,-0.0222,-0.001825));
#5868=CARTESIAN_POINT('Origin',(0.05755,-0.0222,0.043125));
#5869=CARTESIAN_POINT('',(0.05755,-0.0222,0.048125));
#5870=CARTESIAN_POINT('Origin',(0.06655,-0.0222,0.053125));
#6305=UNCERTAINTY_MEASURE_WITH_UNIT(LENGTH_MEASURE(1.E-5),#6349,
'DISTANCE_ACCURACY_VALUE',
'Maximum model space distance between geometric entities at asserted c
onnectivities');
#6323=UNCERTAINTY_MEASURE_WITH_UNIT(LENGTH_MEASURE(1.E-5),#6349,
'DISTANCE_ACCURACY_VALUE',
'Maximum model space distance between geometric entities at asserted c
onnectivities');
#6330=(
GEOMETRIC_REPRESENTATION_CONTEXT(3)
GLOBAL_UNCERTAINTY_ASSIGNED_CONTEXT((#6305))
GLOBAL_UNIT_ASSIGNED_CONTEXT((#6349,#6350,#6351))
REPRESENTATION_CONTEXT('','3D')
);
#6348=(
GEOMETRIC_REPRESENTATION_CONTEXT(3)
GLOBAL_UNCERTAINTY_ASSIGNED_CONTEXT((#6323))
GLOBAL_UNIT_ASSIGNED_CONTEXT((#6349,#6350,#6351))
REPRESENTATION_CONTEXT('','3D')
);
#6349=(
LENGTH_UNIT()
NAMED_UNIT(*)
SI_UNIT($,.METRE.)
);
#6350=(
NAMED_UNIT(*)
PLANE_ANGLE_UNIT()
SI_UNIT($,.RADIAN.)
);
#6351=(
NAMED_UNIT(*)
SI_UNIT($,.STERADIAN.)
SOLID_ANGLE_UNIT()
);
#6358=SHAPE_DEFINITION_REPRESENTATION(#6382,#6482);
#6382=PRODUCT_DEFINITION_SHAPE('',$,#6507);
#6482=SHAPE_REPRESENTATION('',(#3683),#6330);
#6500=PRODUCT_DEFINITION_CONTEXT('part definition',#6574,'design');
#6507=PRODUCT_DEFINITION('End Cap Right','End Cap Right',#6531,#6500);
#6531=PRODUCT_DEFINITION_FORMATION('',$,#6582);
#6574=APPLICATION_CONTEXT('Managed model based 3d engineering');
#6575=PRODUCT_CONTEXT('part definition',#6574,'mechanical');
#6582=PRODUCT('End Cap Right','End Cap Right',
'LEGAL AND USAGE DISCLAIMER: this Data/Model is provided \X2\201C\X0\A
S IS\X2\201D\X0\ for informational and representational only. It is a 
geometric approximation and is NOT engineered, certified, or guarantee
d for dimensional accuracy, exact tolerances, or production-level prec
ision. Vendor disclaims all implied warranties including fitness for a
 particular purpose. DO NOT USE FOR DIRECT PHYSICAL MANUFACTURING, AUT
OMATED PRODUCTION, OR SAFETY-CRITICAL SYSTEMS without independent engi
neering verification and resolution of any design discrepancies.',(#6575));
#6603=PRESENTATION_STYLE_ASSIGNMENT((#6609));
#6609=SURFACE_STYLE_USAGE(.BOTH.,#6615);
#6615=SURFACE_SIDE_STYLE('',(#6621));
#6621=SURFACE_STYLE_FILL_AREA(#6627);
#6627=FILL_AREA_STYLE('Opaque(137,137,137)',(#6633));
#6633=FILL_AREA_STYLE_COLOUR('Opaque(137,137,137)',#6639);
#6639=COLOUR_RGB('Opaque(137,137,137)',0.537254901960784,0.537254901960784,
0.537254901960784);
ENDSEC;
END-ISO-10303-21;
